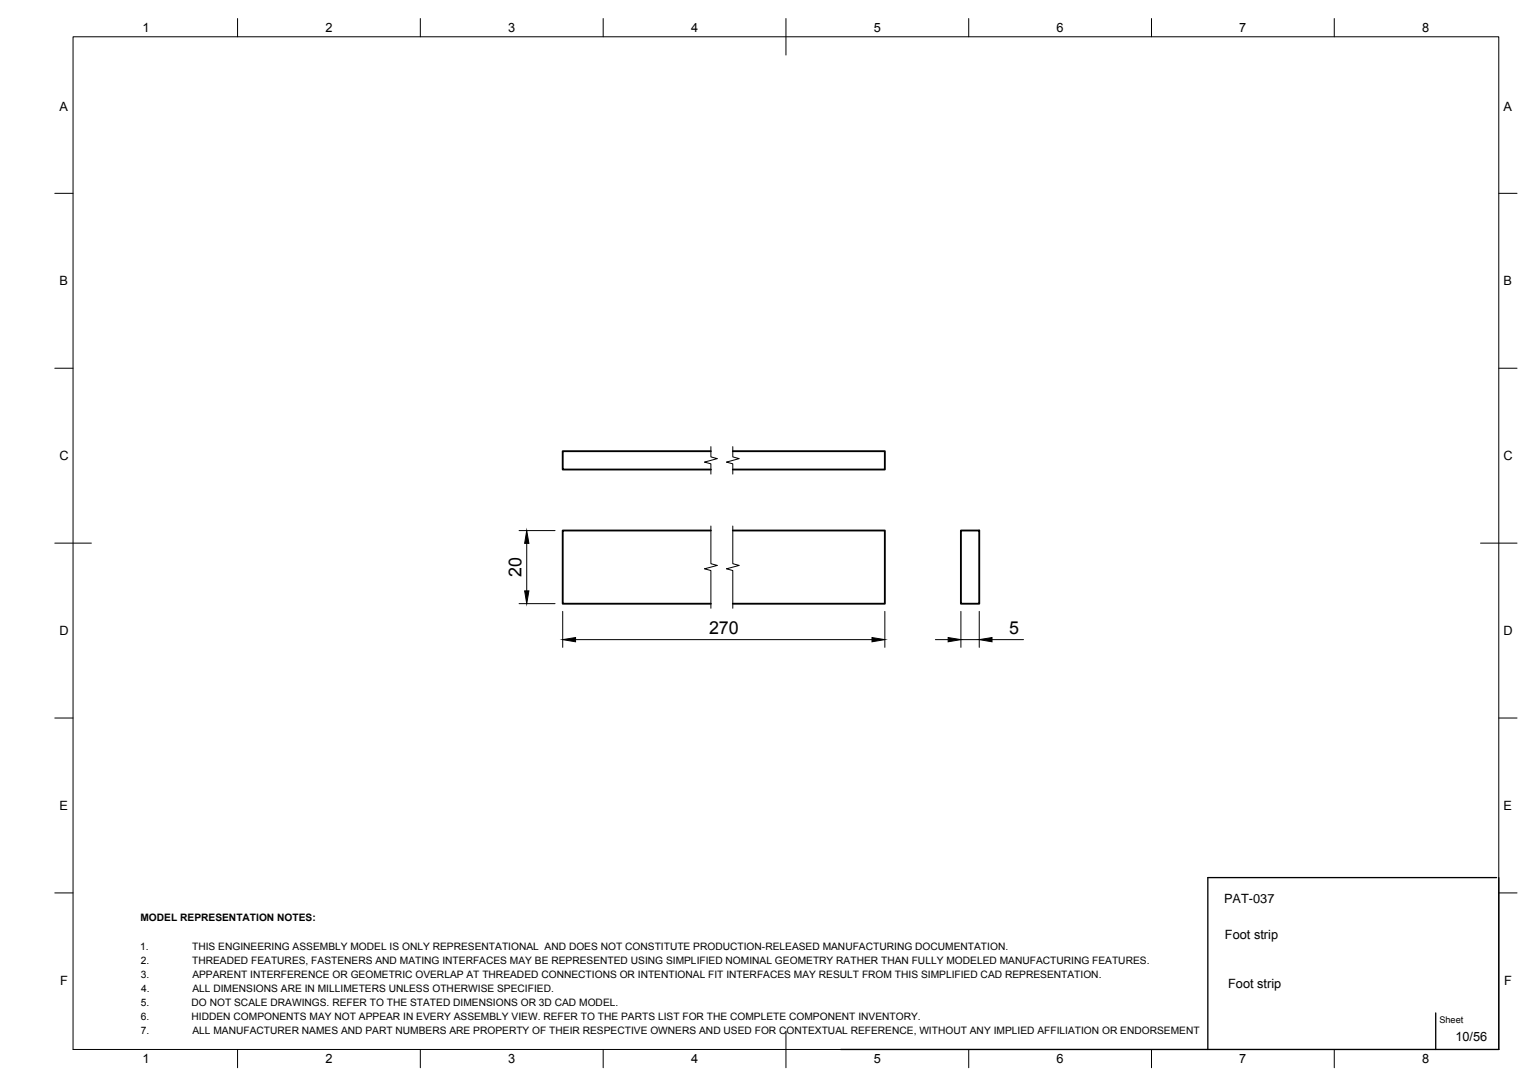
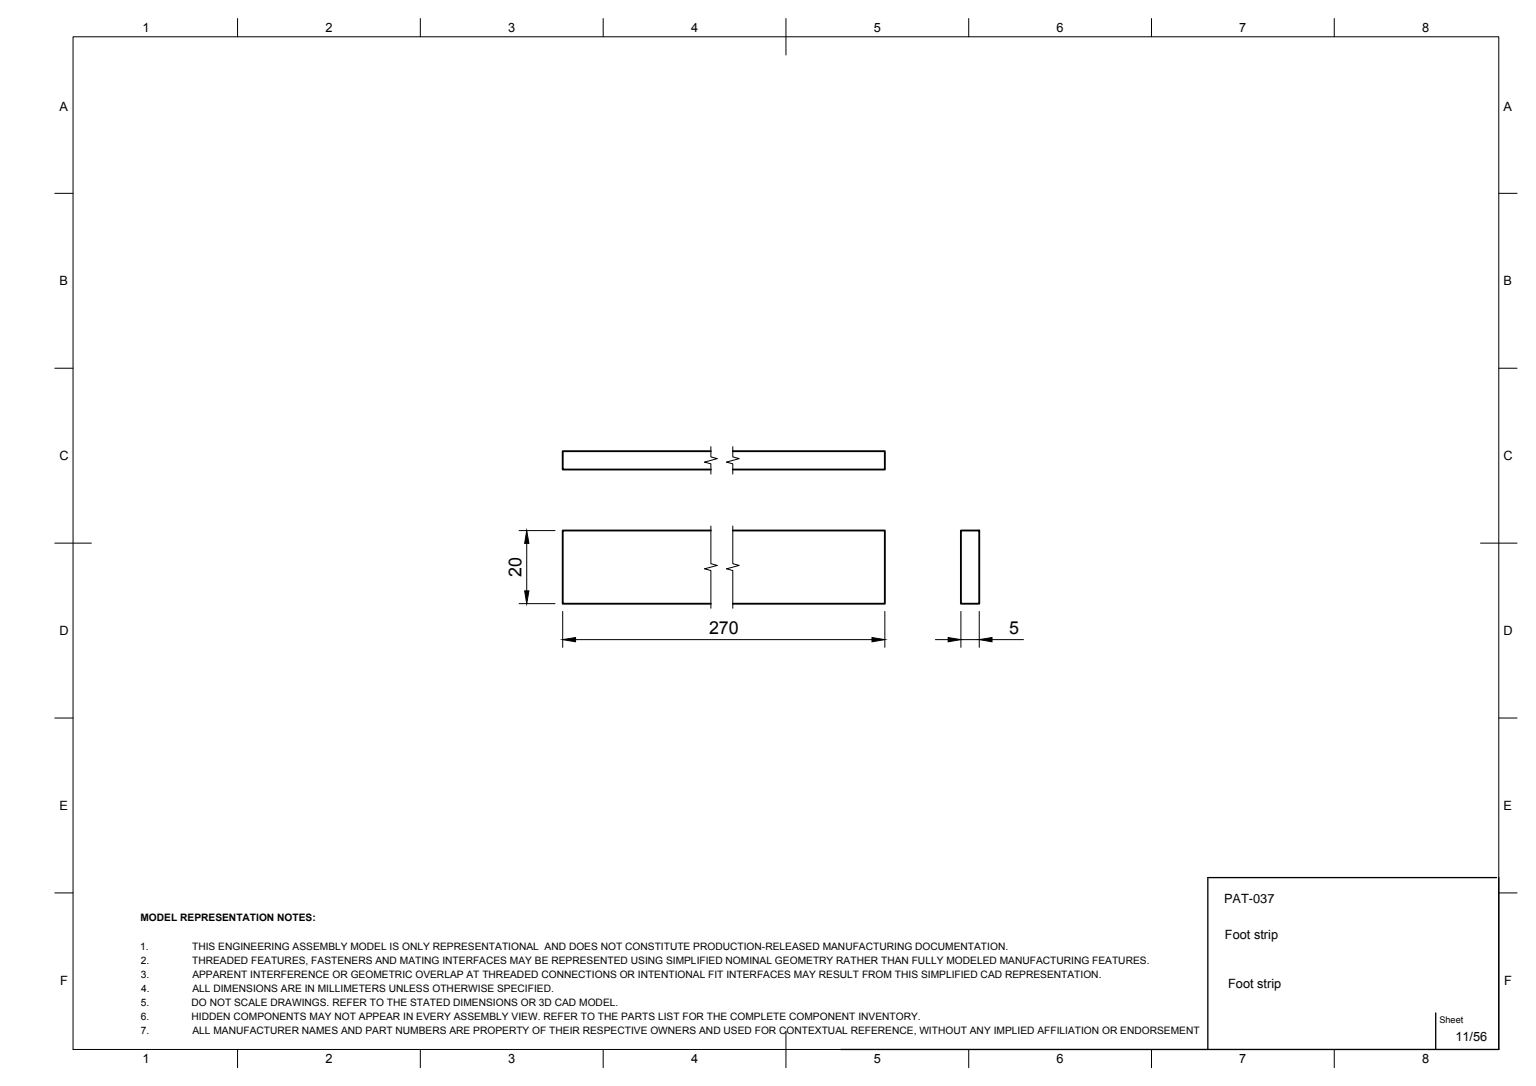
ISO-10303-21;
HEADER;
/* Generated by software containing ST-Developer
 * from STEP Tools, Inc. (www.steptools.com) 
 */

FILE_DESCRIPTION(
/* description */ ('Flywheel Crank-Slider'),
/* implementation_level */ '2;1');

FILE_NAME(
/* name */ 'Foot strip.step',
/* time_stamp */ '2026-10-28T03:23:13-07:00',
/* author */ (''),
/* organization */ (''),
/* preprocessor_version */ 'ST-DEVELOPER v20.2',
/* originating_system */ 'Autodesk Translation Framework v15.17.0.0',
/* authorisation */ '');

FILE_SCHEMA (('AUTOMOTIVE_DESIGN { 1 0 10303 214 3 1 1 }'));
ENDSEC;

DATA;
#10=MECHANICAL_DESIGN_GEOMETRIC_PRESENTATION_REPRESENTATION('',(#677),#17322);
#573=SHAPE_REPRESENTATION_RELATIONSHIP('SRR','None',#17569,#625);
#625=ADVANCED_BREP_SHAPE_REPRESENTATION('',(#738),#17273);
#677=STYLED_ITEM('',(#17917),#738);
#738=MANIFOLD_SOLID_BREP('Body1',#9055);
#1073=PLANE('',#9933);
#1074=PLANE('',#9934);
#1075=PLANE('',#9935);
#1076=PLANE('',#9936);
#1077=PLANE('',#9937);
#1078=PLANE('',#9938);
#1440=FACE_OUTER_BOUND('',#2051,.T.);
#1441=FACE_OUTER_BOUND('',#2052,.T.);
#1442=FACE_OUTER_BOUND('',#2053,.T.);
#1443=FACE_OUTER_BOUND('',#2054,.T.);
#1444=FACE_OUTER_BOUND('',#2055,.T.);
#1445=FACE_OUTER_BOUND('',#2056,.T.);
#2051=EDGE_LOOP('',(#6606,#6607,#6608,#6609));
#2052=EDGE_LOOP('',(#6610,#6611,#6612,#6613));
#2053=EDGE_LOOP('',(#6614,#6615,#6616,#6617));
#2054=EDGE_LOOP('',(#6618,#6619,#6620,#6621));
#2055=EDGE_LOOP('',(#6622,#6623,#6624,#6625));
#2056=EDGE_LOOP('',(#6626,#6627,#6628,#6629));
#2742=LINE('',#14264,#3353);
#2743=LINE('',#14266,#3354);
#2744=LINE('',#14268,#3355);
#2745=LINE('',#14269,#3356);
#2746=LINE('',#14272,#3357);
#2747=LINE('',#14274,#3358);
#2748=LINE('',#14275,#3359);
#2749=LINE('',#14278,#3360);
#2750=LINE('',#14280,#3361);
#2751=LINE('',#14281,#3362);
#2752=LINE('',#14283,#3363);
#2753=LINE('',#14284,#3364);
#3353=VECTOR('',#11454,1.);
#3354=VECTOR('',#11455,1.);
#3355=VECTOR('',#11456,1.);
#3356=VECTOR('',#11457,1.);
#3357=VECTOR('',#11460,1.);
#3358=VECTOR('',#11461,1.);
#3359=VECTOR('',#11462,1.);
#3360=VECTOR('',#11465,1.);
#3361=VECTOR('',#11466,1.);
#3362=VECTOR('',#11467,1.);
#3363=VECTOR('',#11470,1.);
#3364=VECTOR('',#11471,1.);
#4433=VERTEX_POINT('',#14262);
#4434=VERTEX_POINT('',#14263);
#4435=VERTEX_POINT('',#14265);
#4436=VERTEX_POINT('',#14267);
#4437=VERTEX_POINT('',#14271);
#4438=VERTEX_POINT('',#14273);
#4439=VERTEX_POINT('',#14277);
#4440=VERTEX_POINT('',#14279);
#5260=EDGE_CURVE('',#4433,#4434,#2742,.T.);
#5261=EDGE_CURVE('',#4434,#4435,#2743,.T.);
#5262=EDGE_CURVE('',#4436,#4435,#2744,.T.);
#5263=EDGE_CURVE('',#4433,#4436,#2745,.T.);
#5264=EDGE_CURVE('',#4437,#4433,#2746,.T.);
#5265=EDGE_CURVE('',#4438,#4436,#2747,.T.);
#5266=EDGE_CURVE('',#4437,#4438,#2748,.T.);
#5267=EDGE_CURVE('',#4439,#4437,#2749,.T.);
#5268=EDGE_CURVE('',#4440,#4438,#2750,.T.);
#5269=EDGE_CURVE('',#4439,#4440,#2751,.T.);
#5270=EDGE_CURVE('',#4434,#4439,#2752,.T.);
#5271=EDGE_CURVE('',#4435,#4440,#2753,.T.);
#6606=ORIENTED_EDGE('',*,*,#5260,.T.);
#6607=ORIENTED_EDGE('',*,*,#5261,.T.);
#6608=ORIENTED_EDGE('',*,*,#5262,.F.);
#6609=ORIENTED_EDGE('',*,*,#5263,.F.);
#6610=ORIENTED_EDGE('',*,*,#5264,.T.);
#6611=ORIENTED_EDGE('',*,*,#5263,.T.);
#6612=ORIENTED_EDGE('',*,*,#5265,.F.);
#6613=ORIENTED_EDGE('',*,*,#5266,.F.);
#6614=ORIENTED_EDGE('',*,*,#5267,.T.);
#6615=ORIENTED_EDGE('',*,*,#5266,.T.);
#6616=ORIENTED_EDGE('',*,*,#5268,.F.);
#6617=ORIENTED_EDGE('',*,*,#5269,.F.);
#6618=ORIENTED_EDGE('',*,*,#5270,.T.);
#6619=ORIENTED_EDGE('',*,*,#5269,.T.);
#6620=ORIENTED_EDGE('',*,*,#5271,.F.);
#6621=ORIENTED_EDGE('',*,*,#5261,.F.);
#6622=ORIENTED_EDGE('',*,*,#5271,.T.);
#6623=ORIENTED_EDGE('',*,*,#5268,.T.);
#6624=ORIENTED_EDGE('',*,*,#5265,.T.);
#6625=ORIENTED_EDGE('',*,*,#5262,.T.);
#6626=ORIENTED_EDGE('',*,*,#5270,.F.);
#6627=ORIENTED_EDGE('',*,*,#5260,.F.);
#6628=ORIENTED_EDGE('',*,*,#5264,.F.);
#6629=ORIENTED_EDGE('',*,*,#5267,.F.);
#8631=ADVANCED_FACE('',(#1440),#1073,.T.);
#8632=ADVANCED_FACE('',(#1441),#1074,.T.);
#8633=ADVANCED_FACE('',(#1442),#1075,.T.);
#8634=ADVANCED_FACE('',(#1443),#1076,.T.);
#8635=ADVANCED_FACE('',(#1444),#1077,.T.);
#8636=ADVANCED_FACE('',(#1445),#1078,.F.);
#9055=CLOSED_SHELL('',(#8631,#8632,#8633,#8634,#8635,#8636));
#9932=AXIS2_PLACEMENT_3D('',#14260,#11450,#11451);
#9933=AXIS2_PLACEMENT_3D('',#14261,#11452,#11453);
#9934=AXIS2_PLACEMENT_3D('',#14270,#11458,#11459);
#9935=AXIS2_PLACEMENT_3D('',#14276,#11463,#11464);
#9936=AXIS2_PLACEMENT_3D('',#14282,#11468,#11469);
#9937=AXIS2_PLACEMENT_3D('',#14285,#11472,#11473);
#9938=AXIS2_PLACEMENT_3D('',#14286,#11474,#11475);
#11450=DIRECTION('axis',(0.,0.,1.));
#11451=DIRECTION('refdir',(1.,0.,0.));
#11452=DIRECTION('center_axis',(0.,1.,0.));
#11453=DIRECTION('ref_axis',(-1.,0.,0.));
#11454=DIRECTION('',(-1.,0.,0.));
#11455=DIRECTION('',(0.,0.,1.));
#11456=DIRECTION('',(-1.,0.,0.));
#11457=DIRECTION('',(0.,0.,1.));
#11458=DIRECTION('center_axis',(1.,0.,0.));
#11459=DIRECTION('ref_axis',(0.,1.,0.));
#11460=DIRECTION('',(0.,1.,0.));
#11461=DIRECTION('',(0.,1.,0.));
#11462=DIRECTION('',(0.,0.,1.));
#11463=DIRECTION('center_axis',(0.,-1.,0.));
#11464=DIRECTION('ref_axis',(1.,0.,0.));
#11465=DIRECTION('',(1.,0.,0.));
#11466=DIRECTION('',(1.,0.,0.));
#11467=DIRECTION('',(0.,0.,1.));
#11468=DIRECTION('center_axis',(-1.,0.,0.));
#11469=DIRECTION('ref_axis',(0.,-1.,0.));
#11470=DIRECTION('',(0.,-1.,0.));
#11471=DIRECTION('',(0.,-1.,0.));
#11472=DIRECTION('center_axis',(0.,0.,1.));
#11473=DIRECTION('ref_axis',(1.,0.,0.));
#11474=DIRECTION('center_axis',(0.,0.,1.));
#11475=DIRECTION('ref_axis',(1.,0.,0.));
#14260=CARTESIAN_POINT('',(0.,0.,0.));
#14261=CARTESIAN_POINT('Origin',(-6.,9.,-0.5));
#14262=CARTESIAN_POINT('',(-6.,9.,-0.5));
#14263=CARTESIAN_POINT('',(-8.,9.,-0.5));
#14264=CARTESIAN_POINT('',(-6.,9.,-0.5));
#14265=CARTESIAN_POINT('',(-8.,9.,0.));
#14266=CARTESIAN_POINT('',(-8.,9.,-0.5));
#14267=CARTESIAN_POINT('',(-6.,9.,0.));
#14268=CARTESIAN_POINT('',(-6.,9.,0.));
#14269=CARTESIAN_POINT('',(-6.,9.,-0.5));
#14270=CARTESIAN_POINT('Origin',(-6.,-18.,-0.5));
#14271=CARTESIAN_POINT('',(-6.,-18.,-0.5));
#14272=CARTESIAN_POINT('',(-6.,-18.,-0.5));
#14273=CARTESIAN_POINT('',(-6.,-18.,0.));
#14274=CARTESIAN_POINT('',(-6.,-18.,0.));
#14275=CARTESIAN_POINT('',(-6.,-18.,-0.5));
#14276=CARTESIAN_POINT('Origin',(-8.,-18.,-0.5));
#14277=CARTESIAN_POINT('',(-8.,-18.,-0.5));
#14278=CARTESIAN_POINT('',(-8.,-18.,-0.5));
#14279=CARTESIAN_POINT('',(-8.,-18.,0.));
#14280=CARTESIAN_POINT('',(-8.,-18.,0.));
#14281=CARTESIAN_POINT('',(-8.,-18.,-0.5));
#14282=CARTESIAN_POINT('Origin',(-8.,9.,-0.5));
#14283=CARTESIAN_POINT('',(-8.,9.,-0.5));
#14284=CARTESIAN_POINT('',(-8.,9.,0.));
#14285=CARTESIAN_POINT('Origin',(-7.,-4.5,0.));
#14286=CARTESIAN_POINT('Origin',(-7.,-4.5,-0.5));
#17212=UNCERTAINTY_MEASURE_WITH_UNIT(LENGTH_MEASURE(0.001),#17323,
'DISTANCE_ACCURACY_VALUE',
'Maximum model space distance between geometric entities at asserted c
onnectivities');
#17261=UNCERTAINTY_MEASURE_WITH_UNIT(LENGTH_MEASURE(0.001),#17323,
'DISTANCE_ACCURACY_VALUE',
'Maximum model space distance between geometric entities at asserted c
onnectivities');
#17273=(
GEOMETRIC_REPRESENTATION_CONTEXT(3)
GLOBAL_UNCERTAINTY_ASSIGNED_CONTEXT((#17212))
GLOBAL_UNIT_ASSIGNED_CONTEXT((#17323,#17325,#17326))
REPRESENTATION_CONTEXT('','3D')
);
#17322=(
GEOMETRIC_REPRESENTATION_CONTEXT(3)
GLOBAL_UNCERTAINTY_ASSIGNED_CONTEXT((#17261))
GLOBAL_UNIT_ASSIGNED_CONTEXT((#17323,#17325,#17326))
REPRESENTATION_CONTEXT('','3D')
);
#17323=(
LENGTH_UNIT()
NAMED_UNIT(*)
SI_UNIT(.CENTI.,.METRE.)
);
#17325=(
NAMED_UNIT(*)
PLANE_ANGLE_UNIT()
SI_UNIT($,.RADIAN.)
);
#17326=(
NAMED_UNIT(*)
SI_UNIT($,.STERADIAN.)
SOLID_ANGLE_UNIT()
);
#17338=SHAPE_DEFINITION_REPRESENTATION(#17398,#17569);
#17398=PRODUCT_DEFINITION_SHAPE('',$,#17630);
#17569=SHAPE_REPRESENTATION('',(#9932),#17273);
#17618=PRODUCT_DEFINITION_CONTEXT('part definition',#17800,'design');
#17630=PRODUCT_DEFINITION('Foot strip','Foot strip',#17690,#17618);
#17690=PRODUCT_DEFINITION_FORMATION('',$,#17813);
#17800=APPLICATION_CONTEXT(
'Core Data for Automotive Mechanical Design Process');
#17801=PRODUCT_CONTEXT('part definition',#17800,'mechanical');
#17813=PRODUCT('Foot strip','Foot strip','Foot strip',(#17801));
#17911=COLOUR_RGB('Light Blue',0.38,0.62,0.78);
#17912=FILL_AREA_STYLE_COLOUR('',#17911);
#17913=FILL_AREA_STYLE('',(#17912));
#17914=SURFACE_STYLE_FILL_AREA(#17913);
#17915=SURFACE_SIDE_STYLE('',(#17914));
#17916=SURFACE_STYLE_USAGE(.BOTH.,#17915);
#17917=PRESENTATION_STYLE_ASSIGNMENT((#17916));
ENDSEC;
END-ISO-10303-21;
